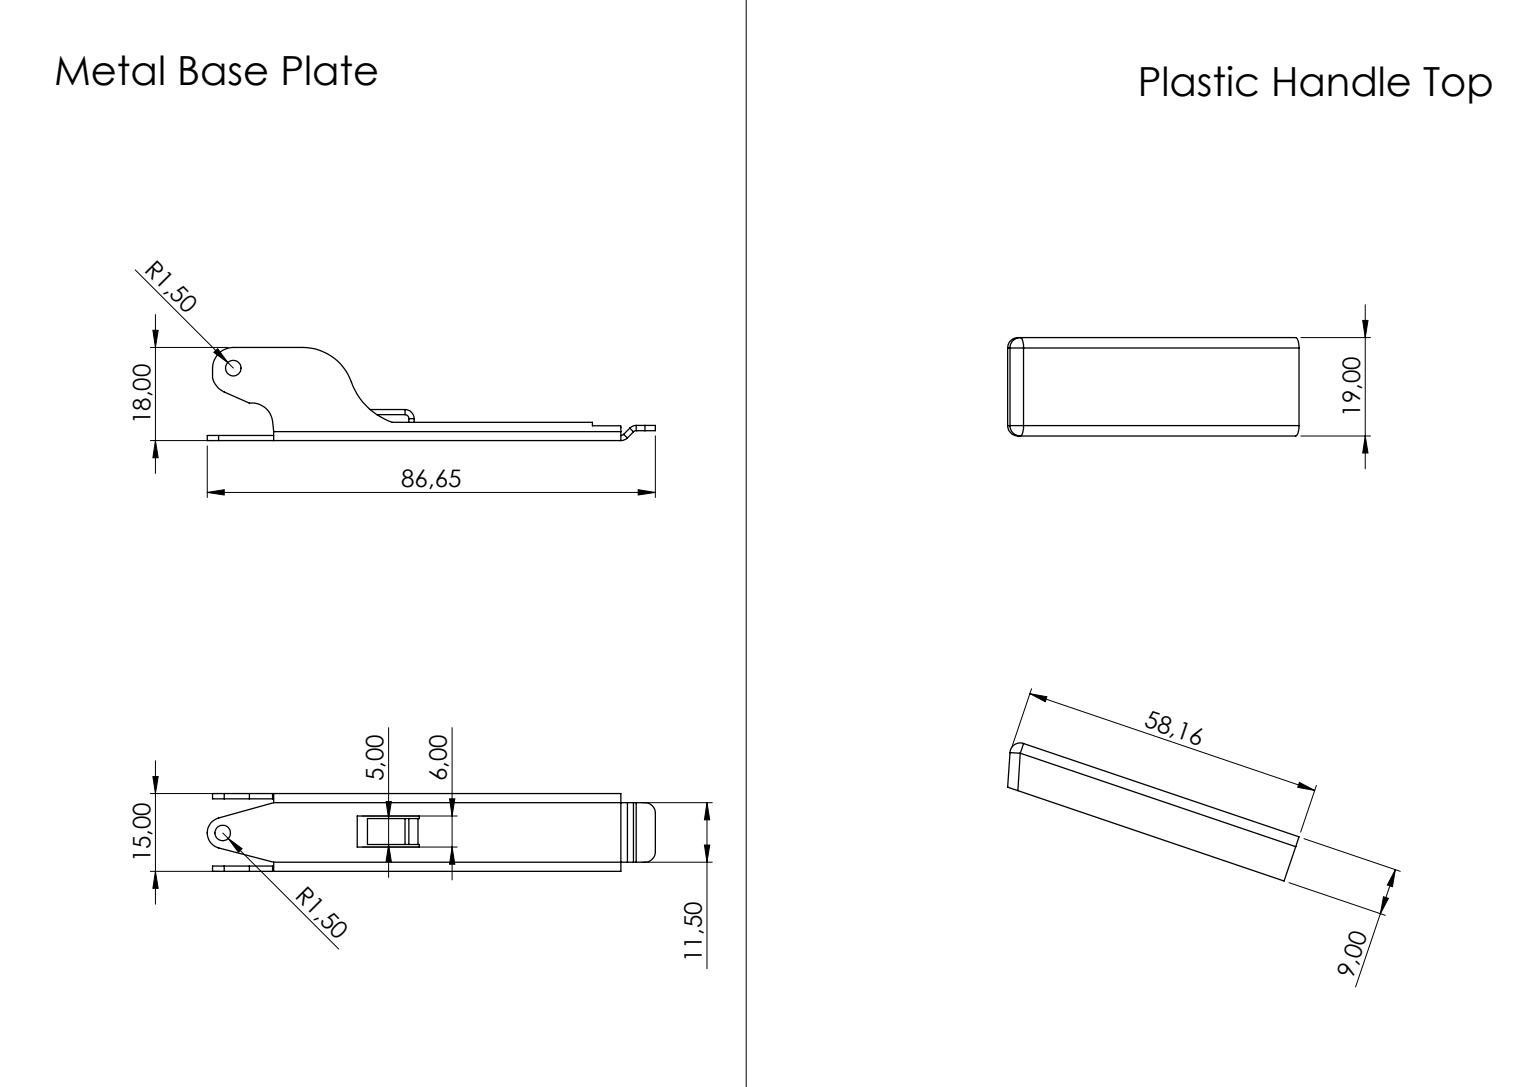
ISO-10303-21;
HEADER;
FILE_DESCRIPTION (('STEP AP214'),
    '1' );
FILE_NAME ('Plastic Handle Top.step',
    '2026-10-06T10:23:46',
    ( '' ),
    ( '' ),
    'SwSTEP 2.0',
    'SolidWorks 2020',
    '' );
FILE_SCHEMA (( 'AUTOMOTIVE_DESIGN' ));
ENDSEC;

DATA;
#49=EDGE_LOOP ( 'NONE', ( #5787, #14617, #11097, #246 ) ) ;
#69=FACE_OUTER_BOUND ( 'NONE', #11931, .T. ) ;
#71=VECTOR ( 'NONE', #6423, 1000.000000000000227 ) ;
#106=ADVANCED_FACE ( 'NONE', ( #10603 ), #18707, .F. ) ;
#219=ORIENTED_EDGE ( 'NONE', *, *, #5616, .T. ) ;
#246=ORIENTED_EDGE ( 'NONE', *, *, #17263, .T. ) ;
#258=ADVANCED_FACE ( 'NONE', ( #25369 ), #5308, .T. ) ;
#299=LINE ( 'NONE', #10238, #21343 ) ;
#343=CARTESIAN_POINT ( 'NONE',  ( 45.81606138205698642, -7.197381196808444237, -3.552044091124070491 ) ) ;
#348=EDGE_CURVE ( 'NONE', #23547, #5555, #499, .T. ) ;
#362=DIRECTION ( 'NONE',  ( -2.385244779468109755E-15, 1.000000000000000000, 0.000000000000000000 ) ) ;
#417=CARTESIAN_POINT ( 'NONE',  ( 30.81606138205696155, 1.773964314019527588, -3.427682652428149623 ) ) ;
#434=ORIENTED_EDGE ( 'NONE', *, *, #3015, .T. ) ;
#447=CARTESIAN_POINT ( 'NONE',  ( 3.816061382056971762, -5.229446354161006560, -9.573232046949398111 ) ) ;
#499=LINE ( 'NONE', #627, #16776 ) ;
#526=AXIS2_PLACEMENT_3D ( 'NONE', #704, #5104, #14630 ) ;
#534=STYLED_ITEM ( 'NONE', ( #16830 ), #19676 ) ;
#560=AXIS2_PLACEMENT_3D ( 'NONE', #2943, #9027, #8898 ) ;
#575=DIRECTION ( 'NONE',  ( 1.000000000000000000, 2.440719103442460911E-15, 1.328886038262200866E-15 ) ) ;
#616=LINE ( 'NONE', #20345, #10667 ) ;
#627=CARTESIAN_POINT ( 'NONE',  ( 29.71606138205698500, -6.548589660139427338, -8.069948661059612505 ) ) ;
#631=CARTESIAN_POINT ( 'NONE',  ( 28.81606138205695444, -23.19619402982950263, 47.16846523730000484 ) ) ;
#704=CARTESIAN_POINT ( 'NONE',  ( 45.81606138205697221, -4.589472609077215104, -6.350807634294793225 ) ) ;
#750=VECTOR ( 'NONE', #17336, 1000.000000000000227 ) ;
#847=ORIENTED_EDGE ( 'NONE', *, *, #24054, .T. ) ;
#862=AXIS2_PLACEMENT_3D ( 'NONE', #7436, #23134, #19536 ) ;
#868=VERTEX_POINT ( 'NONE', #20952 ) ;
#878=CIRCLE ( 'NONE', #9556, 2.000000000000000888 ) ;
#921=CYLINDRICAL_SURFACE ( 'NONE', #3999, 1.100000000000000311 ) ;
#955=FACE_OUTER_BOUND ( 'NONE', #12125, .T. ) ;
#971=SHAPE_REPRESENTATION_RELATIONSHIP ( 'NONE' , 'NONE' ,  #9445, #19676 ) ;
#988=DIRECTION ( 'NONE',  ( -4.040217218240261171E-16, -0.4425581086832399702, 0.8967398287344627850 ) ) ;
#1046=DIRECTION ( 'NONE',  ( -2.727049986597863807E-15, 0.7516416929448760387, 0.6595716529892418079 ) ) ;
#1144=DIRECTION ( 'NONE',  ( 2.727049986597864201E-15, -0.7516416929448760387, -0.6595716529892418079 ) ) ;
#1189=EDGE_CURVE ( 'NONE', #17007, #11300, #6517, .T. ) ;
#1223=PLANE ( 'NONE',  #24789 ) ;
#1237=ORIENTED_EDGE ( 'NONE', *, *, #24724, .T. ) ;
#1291=CARTESIAN_POINT ( 'NONE',  ( 46.91606138205697363, -29.47337283097070681, 44.07055847651734837 ) ) ;
#1309=( LENGTH_UNIT ( ) NAMED_UNIT ( * ) SI_UNIT ( .MILLI., .METRE. ) );
#1431=VECTOR ( 'NONE', #1046, 1000.000000000000000 ) ;
#1439=( NAMED_UNIT ( * ) SI_UNIT ( $, .STERADIAN. ) SOLID_ANGLE_UNIT ( ) );
#1466=ADVANCED_FACE ( 'NONE', ( #21311 ), #19623, .F. ) ;
#1703=DIRECTION ( 'NONE',  ( -1.000000000000000000, -2.411023719125726758E-15, -1.389056744264227588E-15 ) ) ;
#1720=DIRECTION ( 'NONE',  ( -1.000000000000000000, -2.556434596176347380E-15, -1.460819769243627131E-15 ) ) ;
#1767=ORIENTED_EDGE ( 'NONE', *, *, #23665, .F. ) ;
#1771=( LENGTH_UNIT ( ) NAMED_UNIT ( * ) SI_UNIT ( .MILLI., .METRE. ) );
#1792=LINE ( 'NONE', #17788, #13583 ) ;
#1807=AXIS2_PLACEMENT_3D ( 'NONE', #21939, #14085, #12169 ) ;
#1879=PLANE ( 'NONE',  #4650 ) ;
#1958=VERTEX_POINT ( 'NONE', #16654 ) ;
#1977=EDGE_LOOP ( 'NONE', ( #14482, #18335, #5715, #7299 ) ) ;
#2000=AXIS2_PLACEMENT_3D ( 'NONE', #9286, #12766, #22537 ) ;
#2001=EDGE_CURVE ( 'NONE', #5682, #24395, #7833, .T. ) ;
#2034=DIRECTION ( 'NONE',  ( -1.156482317317872465E-16, -0.4425581086832399702, 0.8967398287344626739 ) ) ;
#2126=DIRECTION ( 'NONE',  ( 1.156482317317872711E-16, 0.4425581086832400257, -0.8967398287344628960 ) ) ;
#2251=CARTESIAN_POINT ( 'NONE',  ( 28.81606138205696155, 0.8576245772853319238, -1.570935883000529332 ) ) ;
#2255=EDGE_LOOP ( 'NONE', ( #4585, #7218, #14724, #219 ) ) ;
#2277=EDGE_LOOP ( 'NONE', ( #12064, #434, #20219 ) ) ;
#2401=VERTEX_POINT ( 'NONE', #417 ) ;
#2435=AXIS2_PLACEMENT_3D ( 'NONE', #23279, #13502, #23400 ) ;
#2456=DIRECTION ( 'NONE',  ( 0.000000000000000000, 0.4425581086832397482, -0.8967398287344626739 ) ) ;
#2489=AXIS2_PLACEMENT_3D ( 'NONE', #19390, #23374, #13359 ) ;
#2494=DIRECTION ( 'NONE',  ( -1.786044098272412642E-16, -0.4425581086832399702, 0.8967398287344628960 ) ) ;
#2543=APPLICATION_CONTEXT ( 'automotive_design' ) ;
#2606=EDGE_LOOP ( 'NONE', ( #14663, #13840, #20351 ) ) ;
#2613=DIRECTION ( 'NONE',  ( -1.156482317317870739E-16, -0.4425581086832400257, 0.8967398287344628960 ) ) ;
#2618=CARTESIAN_POINT ( 'NONE',  ( 3.816061382056946449, 1.361611432489073570, -2.592146606185760316 ) ) ;
#2803=ORIENTED_EDGE ( 'NONE', *, *, #5814, .F. ) ;
#2813=ORIENTED_EDGE ( 'NONE', *, *, #19782, .F. ) ;
#2821=DIRECTION ( 'NONE',  ( -2.727049986597864201E-15, 0.7516416929448760387, 0.6595716529892418079 ) ) ;
#2824=FACE_OUTER_BOUND ( 'NONE', #2255, .T. ) ;
#2838=ORIENTED_EDGE ( 'NONE', *, *, #6174, .T. ) ;
#2924=EDGE_CURVE ( 'NONE', #12220, #11300, #22115, .T. ) ;
#2943=CARTESIAN_POINT ( 'NONE',  ( 47.81606138205695089, -23.19619402982945644, 47.16846523730003327 ) ) ;
#2950=LINE ( 'NONE', #24581, #21507 ) ;
#2969=VERTEX_POINT ( 'NONE', #12020 ) ;
#2972=CARTESIAN_POINT ( 'NONE',  ( 45.81606138205697221, -4.589472609077215104, -6.350807634294793225 ) ) ;
#2995=VECTOR ( 'NONE', #19543, 1000.000000000000227 ) ;
#3001=DIRECTION ( 'NONE',  ( 1.156482317317872711E-16, 0.4425581086832400257, -0.8967398287344628960 ) ) ;
#3015=EDGE_CURVE ( 'NONE', #3872, #13887, #6580, .T. ) ;
#3111=ADVANCED_FACE ( 'NONE', ( #2824 ), #6704, .T. ) ;
#3113=EDGE_CURVE ( 'NONE', #3872, #15753, #9022, .T. ) ;
#3213=DIRECTION ( 'NONE',  ( 2.776799322558808202E-15, -0.8967398287344627850, -0.4425581086832400257 ) ) ;
#3290=CARTESIAN_POINT ( 'NONE',  ( 47.81606138205697221, -29.47337283097070326, 44.07055847651734837 ) ) ;
#3426=( NAMED_UNIT ( * ) PLANE_ANGLE_UNIT ( ) SI_UNIT ( $, .RADIAN. ) );
#3490=ORIENTED_EDGE ( 'NONE', *, *, #19731, .F. ) ;
#3623=VECTOR ( 'NONE', #1720, 1000.000000000000000 ) ;
#3643=ORIENTED_EDGE ( 'NONE', *, *, #24491, .F. ) ;
#3644=LINE ( 'NONE', #21431, #13349 ) ;
#3650=DIRECTION ( 'NONE',  ( 2.727049986597864201E-15, -0.7516416929448760387, -0.6595716529892418079 ) ) ;
#3715=CARTESIAN_POINT ( 'NONE',  ( 45.81606138205697221, -4.589472609077215992, -6.350807634294793225 ) ) ;
#3781=AXIS2_PLACEMENT_3D ( 'NONE', #12203, #6014, #18125 ) ;
#3854=EDGE_CURVE ( 'NONE', #8842, #21203, #13959, .T. ) ;
#3866=DIRECTION ( 'NONE',  ( 1.000000000000000000, 2.452751524064190075E-15, 1.339444584486322859E-15 ) ) ;
#3872=VERTEX_POINT ( 'NONE', #5410 ) ;
#3908=CARTESIAN_POINT ( 'NONE',  ( 45.81606138205697931, -6.382952266546141118, -7.235923851661270945 ) ) ;
#3948=CYLINDRICAL_SURFACE ( 'NONE', #22674, 2.000000000000000888 ) ;
#3979=CARTESIAN_POINT ( 'NONE',  ( 30.81606138205697931, -4.589472609077251519, -6.350807634294812765 ) ) ;
#3994=ORIENTED_EDGE ( 'NONE', *, *, #7465, .F. ) ;
#3999=AXIS2_PLACEMENT_3D ( 'NONE', #7120, #14975, #22831 ) ;
#4000=ORIENTED_EDGE ( 'NONE', *, *, #23645, .T. ) ;
#4031=CARTESIAN_POINT ( 'NONE',  ( 28.81606138205695089, 1.394403967322826121, -2.658592958638802184 ) ) ;
#4078=PLANE ( 'NONE',  #21448 ) ;
#4099=ORIENTED_EDGE ( 'NONE', *, *, #4913, .F. ) ;
#4178=ORIENTED_EDGE ( 'NONE', *, *, #14604, .F. ) ;
#4203=CARTESIAN_POINT ( 'NONE',  ( 30.81606138205697931, -6.210967385200574675, -3.065230171572521645 ) ) ;
#4382=LINE ( 'NONE', #12626, #24258 ) ;
#4391=ADVANCED_FACE ( 'NONE', ( #24886 ), #16796, .F. ) ;
#4431=AXIS2_PLACEMENT_3D ( 'NONE', #2972, #8802, #18454 ) ;
#4512=CIRCLE ( 'NONE', #2435, 1.100000000000000311 ) ;
#4533=CARTESIAN_POINT ( 'NONE',  ( 45.81606138205695089, 1.361611432489176821, -2.592146606185703916 ) ) ;
#4570=VECTOR ( 'NONE', #11563, 1000.000000000000227 ) ;
#4585=ORIENTED_EDGE ( 'NONE', *, *, #5809, .T. ) ;
#4633=UNCERTAINTY_MEASURE_WITH_UNIT (LENGTH_MEASURE( 1.000000000000000082E-05 ), #1771, 'distance_accuracy_value', 'NONE');
#4640=ORIENTED_EDGE ( 'NONE', *, *, #17576, .F. ) ;
#4650=AXIS2_PLACEMENT_3D ( 'NONE', #15290, #5515, #15164 ) ;
#4717=PRODUCT_DEFINITION_FORMATION_WITH_SPECIFIED_SOURCE ( 'ANY', '', #11362, .NOT_KNOWN. ) ;
#4791=CARTESIAN_POINT ( 'NONE',  ( 3.816061382056972207, -3.863943790789065691, -7.177613496534135606 ) ) ;
#4913=EDGE_CURVE ( 'NONE', #868, #2401, #16899, .T. ) ;
#4966=EDGE_LOOP ( 'NONE', ( #17447, #12628, #13369, #10650 ) ) ;
#4984=DIRECTION ( 'NONE',  ( 1.000000000000000000, 2.440719103442461700E-15, 1.328886038262201260E-15 ) ) ;
#5024=AXIS2_PLACEMENT_3D ( 'NONE', #25467, #7595, #12106 ) ;
#5031=CARTESIAN_POINT ( 'NONE',  ( 2.480162969315272434E-14, -8.004447042669575296, -3.950346388939042885 ) ) ;
#5035=ORIENTED_EDGE ( 'NONE', *, *, #24912, .F. ) ;
#5104=DIRECTION ( 'NONE',  ( 1.493079894517851385E-15, 0.4425581086832399147, -0.8967398287344626739 ) ) ;
#5119=ORIENTED_EDGE ( 'NONE', *, *, #22759, .F. ) ;
#5125=ORIENTED_EDGE ( 'NONE', *, *, #5616, .F. ) ;
#5132=DIRECTION ( 'NONE',  ( 0.000000000000000000, -0.8967398287344627850, -0.4425581086832399702 ) ) ;
#5163=ORIENTED_EDGE ( 'NONE', *, *, #10385, .F. ) ;
#5200=FACE_OUTER_BOUND ( 'NONE', #18200, .T. ) ;
#5234=CARTESIAN_POINT ( 'NONE',  ( 45.81606138205695089, 1.773964314019564448, -3.427682652428129195 ) ) ;
#5308=PLANE ( 'NONE',  #13883 ) ;
#5352=ORIENTED_EDGE ( 'NONE', *, *, #6293, .T. ) ;
#5410=CARTESIAN_POINT ( 'NONE',  ( 47.81606138205697931, -4.589472609077211551, -6.350807634294790560 ) ) ;
#5422=ORIENTED_EDGE ( 'NONE', *, *, #23086, .F. ) ;
#5427=ORIENTED_EDGE ( 'NONE', *, *, #3113, .T. ) ;
#5515=DIRECTION ( 'NONE',  ( 6.109829820097539848E-16, -0.6595716529892418079, 0.7516416929448760387 ) ) ;
#5555=VERTEX_POINT ( 'NONE', #12516 ) ;
#5576=SHAPE_DEFINITION_REPRESENTATION ( #25327, #9445 ) ;
#5616=EDGE_CURVE ( 'NONE', #13887, #14165, #23652, .T. ) ;
#5677=ORIENTED_EDGE ( 'NONE', *, *, #20745, .T. ) ;
#5682=VERTEX_POINT ( 'NONE', #11946 ) ;
#5715=ORIENTED_EDGE ( 'NONE', *, *, #348, .T. ) ;
#5732=VECTOR ( 'NONE', #11228, 1000.000000000000000 ) ;
#5734=DIRECTION ( 'NONE',  ( 0.000000000000000000, 0.4425581086832399702, -0.8967398287344626739 ) ) ;
#5782=VECTOR ( 'NONE', #23672, 1000.000000000000000 ) ;
#5787=ORIENTED_EDGE ( 'NONE', *, *, #9395, .T. ) ;
#5809=EDGE_CURVE ( 'NONE', #14165, #19639, #14493, .T. ) ;
#5814=EDGE_CURVE ( 'NONE', #24859, #20881, #21850, .T. ) ;
#5834=FACE_OUTER_BOUND ( 'NONE', #13508, .T. ) ;
#5968=EDGE_LOOP ( 'NONE', ( #20132, #9383, #11486, #17134 ) ) ;
#5992=CARTESIAN_POINT ( 'NONE',  ( 30.81606138205697931, -3.863943790789087895, -7.177613496534175574 ) ) ;
#6012=DIRECTION ( 'NONE',  ( 0.000000000000000000, 0.8967398287344626739, 0.4425581086832399147 ) ) ;
#6014=DIRECTION ( 'NONE',  ( 1.000000000000000000, 2.490066548941357028E-15, 1.228895056384528999E-15 ) ) ;
#6033=CARTESIAN_POINT ( 'NONE',  ( 45.81606138205697931, -6.548589660139387369, -8.069948661059591188 ) ) ;
#6125=CARTESIAN_POINT ( 'NONE',  ( 45.81606138205697931, -30.45978664257862434, 43.58374455696579730 ) ) ;
#6174=EDGE_CURVE ( 'NONE', #24859, #17007, #3644, .T. ) ;
#6214=ADVANCED_FACE ( 'NONE', ( #16378 ), #12291, .T. ) ;
#6256=ORIENTED_EDGE ( 'NONE', *, *, #14050, .T. ) ;
#6293=EDGE_CURVE ( 'NONE', #21203, #12220, #22317, .T. ) ;
#6350=EDGE_CURVE ( 'NONE', #9234, #24670, #24355, .T. ) ;
#6354=ORIENTED_EDGE ( 'NONE', *, *, #2001, .T. ) ;
#6397=AXIS2_PLACEMENT_3D ( 'NONE', #21913, #8519, #18058 ) ;
#6417=EDGE_CURVE ( 'NONE', #3872, #5682, #24603, .T. ) ;
#6423=DIRECTION ( 'NONE',  ( -0.000000000000000000, -0.4425581086832399702, 0.8967398287344626739 ) ) ;
#6446=DIRECTION ( 'NONE',  ( 2.727049986597864201E-15, -0.7516416929448760387, -0.6595716529892418079 ) ) ;
#6464=AXIS2_PLACEMENT_3D ( 'NONE', #9572, #25251, #19726 ) ;
#6501=ORIENTED_EDGE ( 'NONE', *, *, #5814, .T. ) ;
#6517=LINE ( 'NONE', #16422, #18384 ) ;
#6580=CIRCLE ( 'NONE', #9890, 2.000000000000000000 ) ;
#6682=ORIENTED_EDGE ( 'NONE', *, *, #3854, .F. ) ;
#6704=PLANE ( 'NONE',  #15985 ) ;
#6738=DIRECTION ( 'NONE',  ( -1.156482317317870739E-16, -0.4425581086832400257, 0.8967398287344628960 ) ) ;
#6883=VERTEX_POINT ( 'NONE', #7078 ) ;
#7031=FACE_OUTER_BOUND ( 'NONE', #20181, .T. ) ;
#7075=EDGE_CURVE ( 'NONE', #13774, #2969, #9534, .T. ) ;
#7078=CARTESIAN_POINT ( 'NONE',  ( 45.81606138205698642, -5.575886420685123745, -6.837621553846354949 ) ) ;
#7108=CARTESIAN_POINT ( 'NONE',  ( 30.81606138205696155, 1.773964314019528477, -3.427682652428150067 ) ) ;
#7113=CARTESIAN_POINT ( 'NONE',  ( 47.81606138205695800, 0.4548210080410876599, -1.924399266538374009 ) ) ;
#7120=CARTESIAN_POINT ( 'NONE',  ( 45.81606138205697931, -6.548589660139387369, -8.069948661059591188 ) ) ;
#7135=EDGE_CURVE ( 'NONE', #5555, #20798, #11592, .T. ) ;
#7145=ORIENTED_EDGE ( 'NONE', *, *, #17263, .F. ) ;
#7163=DIRECTION ( 'NONE',  ( 1.156482317317870492E-16, 0.4425581086832399702, -0.8967398287344626739 ) ) ;
#7206=ORIENTED_EDGE ( 'NONE', *, *, #20424, .T. ) ;
#7215=CARTESIAN_POINT ( 'NONE',  ( 46.91606138205695231, -23.19619402982945644, 47.16846523730003327 ) ) ;
#7218=ORIENTED_EDGE ( 'NONE', *, *, #24491, .T. ) ;
#7299=ORIENTED_EDGE ( 'NONE', *, *, #9417, .F. ) ;
#7412=DIRECTION ( 'NONE',  ( 1.000000000000000000, 2.490066548941357423E-15, 1.228895056384527422E-15 ) ) ;
#7435=CARTESIAN_POINT ( 'NONE',  ( 29.71606138205696368, 0.06621141594066179414, 0.03267658921015577367 ) ) ;
#7436=CARTESIAN_POINT ( 'NONE',  ( 30.81606138205697221, -29.47337283097074234, 44.07055847651731995 ) ) ;
#7453=PLANE ( 'NONE',  #15618 ) ;
#7465=EDGE_CURVE ( 'NONE', #9234, #1958, #9990, .T. ) ;
#7472=( GEOMETRIC_REPRESENTATION_CONTEXT ( 3 ) GLOBAL_UNCERTAINTY_ASSIGNED_CONTEXT ( ( #12580 ) ) GLOBAL_UNIT_ASSIGNED_CONTEXT ( ( #1309, #19101, #1439 ) ) REPRESENTATION_CONTEXT ( 'NONE', 'WORKASPACE' ) );
#7549=LINE ( 'NONE', #15400, #3623 ) ;
#7595=DIRECTION ( 'NONE',  ( -1.786044098272412642E-16, -0.4425581086832399702, 0.8967398287344628960 ) ) ;
#7650=EDGE_LOOP ( 'NONE', ( #11210, #5427, #18516, #21243 ) ) ;
#7654=ORIENTED_EDGE ( 'NONE', *, *, #14473, .F. ) ;
#7695=EDGE_CURVE ( 'NONE', #868, #9234, #878, .T. ) ;
#7770=ADVANCED_FACE ( 'NONE', ( #22444 ), #10260, .F. ) ;
#7833=( BOUNDED_CURVE ( )  B_SPLINE_CURVE ( 3, ( #13430, #15352, #11376, #13182 ),
 .UNSPECIFIED., .F., .T. ) 
 B_SPLINE_CURVE_WITH_KNOTS ( ( 4, 4 ),
 ( 1.570796326794895004, 3.141592653589793116 ),
 .UNSPECIFIED. ) 
 CURVE ( )  GEOMETRIC_REPRESENTATION_ITEM ( )  RATIONAL_B_SPLINE_CURVE ( ( 1.000000000000000000, 0.8047378541243646044, 0.8047378541243646044, 1.000000000000000000 ) ) 
 REPRESENTATION_ITEM ( '' )  );
#7841=LINE ( 'NONE', #15304, #5782 ) ;
#7872=ORIENTED_EDGE ( 'NONE', *, *, #5809, .F. ) ;
#8002=CYLINDRICAL_SURFACE ( 'NONE', #23442, 2.000000000000000000 ) ;
#8024=DIRECTION ( 'NONE',  ( -1.000000000000000000, -1.497661361212515810E-15, -3.239770556388344395E-15 ) ) ;
#8072=ORIENTED_EDGE ( 'NONE', *, *, #12737, .F. ) ;
#8091=DIRECTION ( 'NONE',  ( -1.000000000000000000, -2.556434596176347380E-15, -1.460819769243627131E-15 ) ) ;
#8096=ORIENTED_EDGE ( 'NONE', *, *, #22081, .F. ) ;
#8228=AXIS2_PLACEMENT_3D ( 'NONE', #10761, #3001, #22848 ) ;
#8268=CIRCLE ( 'NONE', #2489, 2.000000000000000000 ) ;
#8324=DIRECTION ( 'NONE',  ( -1.000000000000000000, -2.556434596176347380E-15, -1.460819769243627131E-15 ) ) ;
#8372=DIRECTION ( 'NONE',  ( 2.792262043613788141E-15, -0.8967398287344626739, -0.4425581086832399147 ) ) ;
#8402=EDGE_CURVE ( 'NONE', #5555, #11300, #16808, .T. ) ;
#8419=ORIENTED_EDGE ( 'NONE', *, *, #14782, .F. ) ;
#8454=ORIENTED_EDGE ( 'NONE', *, *, #7135, .F. ) ;
#8519=DIRECTION ( 'NONE',  ( 1.000000000000000000, 2.452751524064188892E-15, 1.339444584486322859E-15 ) ) ;
#8530=CIRCLE ( 'NONE', #6464, 2.000000000000000000 ) ;
#8607=ORIENTED_EDGE ( 'NONE', *, *, #3854, .T. ) ;
#8645=FACE_OUTER_BOUND ( 'NONE', #49, .T. ) ;
#8802=DIRECTION ( 'NONE',  ( 1.000000000000000000, 2.490066548941357028E-15, 1.228895056384528999E-15 ) ) ;
#8842=VERTEX_POINT ( 'NONE', #24483 ) ;
#8847=VECTOR ( 'NONE', #23855, 1000.000000000000227 ) ;
#8859=FILL_AREA_STYLE ('',( #13773 ) ) ;
#8890=VERTEX_POINT ( 'NONE', #14842 ) ;
#8898=DIRECTION ( 'NONE',  ( -2.452751524064188892E-15, 1.000000000000000000, 0.000000000000000000 ) ) ;
#8899=ADVANCED_FACE ( 'NONE', ( #12928 ), #921, .F. ) ;
#8903=CARTESIAN_POINT ( 'NONE',  ( 28.81606138205698997, -6.548589660139430002, -8.069948661059614281 ) ) ;
#8938=EDGE_CURVE ( 'NONE', #868, #1958, #8530, .T. ) ;
#9022=CIRCLE ( 'NONE', #21755, 2.000000000000000000 ) ;
#9027=DIRECTION ( 'NONE',  ( 1.000000000000000000, 2.452751524064188892E-15, 1.339444584486322859E-15 ) ) ;
#9102=ADVANCED_FACE ( 'NONE', ( #18433 ), #18315, .F. ) ;
#9190=CIRCLE ( 'NONE', #526, 1.099999999999999867 ) ;
#9213=MECHANICAL_DESIGN_GEOMETRIC_PRESENTATION_REPRESENTATION('',(#534),#24807);
#9222=ORIENTED_EDGE ( 'NONE', *, *, #16436, .T. ) ;
#9234=VERTEX_POINT ( 'NONE', #19986 ) ;
#9277=CARTESIAN_POINT ( 'NONE',  ( 28.81606138205695444, -23.19619402982950263, 47.16846523730000484 ) ) ;
#9286=CARTESIAN_POINT ( 'NONE',  ( 0.000000000000000000, 0.000000000000000000, 0.000000000000000000 ) ) ;
#9322=PRESENTATION_STYLE_ASSIGNMENT (( #10985 ) ) ;
#9378=DIRECTION ( 'NONE',  ( 1.156482317317872465E-16, 0.4425581086832399702, -0.8967398287344626739 ) ) ;
#9383=ORIENTED_EDGE ( 'NONE', *, *, #7075, .F. ) ;
#9393=EDGE_LOOP ( 'NONE', ( #8607, #14361, #5163 ) ) ;
#9395=EDGE_CURVE ( 'NONE', #16417, #8890, #2950, .T. ) ;
#9417=EDGE_CURVE ( 'NONE', #12220, #5555, #16146, .T. ) ;
#9438=ORIENTED_EDGE ( 'NONE', *, *, #7135, .T. ) ;
#9445=SHAPE_REPRESENTATION ( 'Plastic Handle Top', ( #2000 ), #20728 ) ;
#9498=CARTESIAN_POINT ( 'NONE',  ( 30.81606138205697931, -5.823060841851313008, -8.896754523299021500 ) ) ;
#9525=AXIS2_PLACEMENT_3D ( 'NONE', #16163, #16541, #12585 ) ;
#9534=LINE ( 'NONE', #15440, #15445 ) ;
#9556=AXIS2_PLACEMENT_3D ( 'NONE', #14000, #19793, #20047 ) ;
#9572=CARTESIAN_POINT ( 'NONE',  ( 30.81606138205697931, -4.589472609077253296, -6.350807634294812765 ) ) ;
#9607=CARTESIAN_POINT ( 'NONE',  ( 30.81606138205698997, -30.45978664257865987, 43.58374455696577598 ) ) ;
#9755=CARTESIAN_POINT ( 'NONE',  ( 45.81606138205697931, -8.004447042669465162, -3.950346388938982045 ) ) ;
#9890=AXIS2_PLACEMENT_3D ( 'NONE', #14816, #18688, #16620 ) ;
#9960=CIRCLE ( 'NONE', #5024, 1.099999999999998312 ) ;
#9969=CARTESIAN_POINT ( 'NONE',  ( 45.81606138205697221, -31.26685248843962839, 43.18544225915087509 ) ) ;
#9990=CIRCLE ( 'NONE', #24358, 1.999999999999999778 ) ;
#10053=EDGE_CURVE ( 'NONE', #18026, #24670, #24929, .T. ) ;
#10056=ADVANCED_FACE ( 'NONE', ( #13754 ), #1879, .T. ) ;
#10059=AXIS2_PLACEMENT_3D ( 'NONE', #14746, #7412, #11149 ) ;
#10098=CARTESIAN_POINT ( 'NONE',  ( 28.81606138205696155, 0.8576245772853319238, -1.570935883000529332 ) ) ;
#10149=CARTESIAN_POINT ( 'NONE',  ( 28.81606138205695444, -23.19619402982950263, 47.16846523730000484 ) ) ;
#10238=CARTESIAN_POINT ( 'NONE',  ( 45.81606138205697931, -5.229446354160903532, -9.573232046949343044 ) ) ;
#10253=EDGE_LOOP ( 'NONE', ( #5035, #11003, #23694, #3643 ) ) ;
#10260=SPHERICAL_SURFACE ( 'NONE', #3781, 1.100000000000000089 ) ;
#10263=ORIENTED_EDGE ( 'NONE', *, *, #6350, .T. ) ;
#10316=DIRECTION ( 'NONE',  ( 1.156482317317871478E-16, 0.4425581086832399702, -0.8967398287344626739 ) ) ;
#10349=FILL_AREA_STYLE_COLOUR ( '', #17355 ) ;
#10370=ORIENTED_EDGE ( 'NONE', *, *, #18072, .F. ) ;
#10385=EDGE_CURVE ( 'NONE', #8842, #6883, #9190, .T. ) ;
#10387=CARTESIAN_POINT ( 'NONE',  ( 3.816061382056966433, -4.589472609077318133, -6.350807634294847404 ) ) ;
#10480=ORIENTED_EDGE ( 'NONE', *, *, #6293, .F. ) ;
#10487=FACE_OUTER_BOUND ( 'NONE', #10973, .T. ) ;
#10495=DIRECTION ( 'NONE',  ( 0.000000000000000000, -0.8967398287344626739, -0.4425581086832399147 ) ) ;
#10581=DIRECTION ( 'NONE',  ( 0.000000000000000000, -0.6595716529892419189, 0.7516416929448759277 ) ) ;
#10603=FACE_OUTER_BOUND ( 'NONE', #9393, .T. ) ;
#10650=ORIENTED_EDGE ( 'NONE', *, *, #17841, .F. ) ;
#10653=ORIENTED_EDGE ( 'NONE', *, *, #8402, .F. ) ;
#10667=VECTOR ( 'NONE', #8372, 1000.000000000000227 ) ;
#10679=AXIS2_PLACEMENT_3D ( 'NONE', #3715, #15570, #25084 ) ;
#10712=DIRECTION ( 'NONE',  ( 0.000000000000000000, 0.6595716529892415858, -0.7516416929448761497 ) ) ;
#10738=SURFACE_STYLE_FILL_AREA ( #18971 ) ;
#10761=CARTESIAN_POINT ( 'NONE',  ( 30.81606138205697931, -6.210967385200574675, -3.065230171572521645 ) ) ;
#10784=LINE ( 'NONE', #18635, #17333 ) ;
#10814=UNCERTAINTY_MEASURE_WITH_UNIT (LENGTH_MEASURE( 1.000000000000000082E-05 ), #24666, 'distance_accuracy_value', 'NONE');
#10852=ORIENTED_EDGE ( 'NONE', *, *, #23357, .T. ) ;
#10865=LINE ( 'NONE', #20781, #12440 ) ;
#10973=EDGE_LOOP ( 'NONE', ( #18626, #21487, #6501, #17423 ) ) ;
#10985=SURFACE_STYLE_USAGE ( .BOTH. , #23073 ) ;
#11003=ORIENTED_EDGE ( 'NONE', *, *, #6350, .F. ) ;
#11064=ORIENTED_EDGE ( 'NONE', *, *, #6174, .F. ) ;
#11090=DIRECTION ( 'NONE',  ( -2.727049986597863807E-15, 0.7516416929448760387, 0.6595716529892418079 ) ) ;
#11097=ORIENTED_EDGE ( 'NONE', *, *, #6417, .T. ) ;
#11149=DIRECTION ( 'NONE',  ( 0.000000000000000000, 0.4425581086832397482, -0.8967398287344626739 ) ) ;
#11169=SURFACE_STYLE_FILL_AREA ( #8859 ) ;
#11200=DIRECTION ( 'NONE',  ( 2.452751524064188892E-15, -1.000000000000000000, 0.000000000000000000 ) ) ;
#11210=ORIENTED_EDGE ( 'NONE', *, *, #6417, .F. ) ;
#11228=DIRECTION ( 'NONE',  ( -2.727049986597863807E-15, 0.7516416929448760387, 0.6595716529892418079 ) ) ;
#11300=VERTEX_POINT ( 'NONE', #19043 ) ;
#11305=CARTESIAN_POINT ( 'NONE',  ( 28.81606138205697576, -29.47337283097074589, 44.07055847651732705 ) ) ;
#11358=ORIENTED_EDGE ( 'NONE', *, *, #22759, .T. ) ;
#11362=PRODUCT ( 'Plastic Handle Top', 'Plastic Handle Top', '', ( #11380 ) ) ;
#11376=CARTESIAN_POINT ( 'NONE',  ( 46.98763425731077348, 1.773964314019564448, -3.427682652428131416 ) ) ;
#11380=PRODUCT_CONTEXT ( 'NONE', #21976, 'mechanical' ) ;
#11416=LINE ( 'NONE', #3290, #750 ) ;
#11486=ORIENTED_EDGE ( 'NONE', *, *, #20745, .F. ) ;
#11550=AXIS2_PLACEMENT_3D ( 'NONE', #6033, #23915, #20192 ) ;
#11563=DIRECTION ( 'NONE',  ( -1.156482317317870492E-16, -0.4425581086832399702, 0.8967398287344626739 ) ) ;
#11592=LINE ( 'NONE', #15182, #25181 ) ;
#11643=VECTOR ( 'NONE', #9378, 1000.000000000000227 ) ;
#11677=FACE_OUTER_BOUND ( 'NONE', #23537, .T. ) ;
#11825=CARTESIAN_POINT ( 'NONE',  ( 45.81606138205697221, -6.210967385200538260, -3.065230171572501661 ) ) ;
#11856=ADVANCED_FACE ( 'NONE', ( #7031 ), #1223, .F. ) ;
#11857=AXIS2_PLACEMENT_3D ( 'NONE', #23358, #3650, #13456 ) ;
#11898=DIRECTION ( 'NONE',  ( 1.000000000000000000, 2.490066548941357423E-15, 1.228895056384527422E-15 ) ) ;
#11931=EDGE_LOOP ( 'NONE', ( #15665, #7206, #14397, #4000 ) ) ;
#11940=LINE ( 'NONE', #9498, #22519 ) ;
#11945=VERTEX_POINT ( 'NONE', #18756 ) ;
#11946=CARTESIAN_POINT ( 'NONE',  ( 47.81606138205695800, 0.8576245772853805516, -1.570935883000508460 ) ) ;
#11949=DIRECTION ( 'NONE',  ( 6.109829820097539848E-16, -0.6595716529892418079, 0.7516416929448760387 ) ) ;
#11974=FACE_OUTER_BOUND ( 'NONE', #7650, .T. ) ;
#12018=STYLED_ITEM ( 'NONE', ( #9322 ), #17206 ) ;
#12020=CARTESIAN_POINT ( 'NONE',  ( 46.91606138205695231, -23.19619402982945644, 47.16846523730003327 ) ) ;
#12030=VECTOR ( 'NONE', #4984, 1000.000000000000000 ) ;
#12064=ORIENTED_EDGE ( 'NONE', *, *, #3113, .F. ) ;
#12106=DIRECTION ( 'NONE',  ( 0.000000000000000000, -0.8967398287344631180, -0.4425581086832393041 ) ) ;
#12125=EDGE_LOOP ( 'NONE', ( #18841, #20828, #24186, #5352 ) ) ;
#12169=DIRECTION ( 'NONE',  ( 0.000000000000000000, 0.6595716529892419189, -0.7516416929448759277 ) ) ;
#12203=CARTESIAN_POINT ( 'NONE',  ( 30.81606138205697931, -4.589472609077253296, -6.350807634294811876 ) ) ;
#12220=VERTEX_POINT ( 'NONE', #5992 ) ;
#12279=CARTESIAN_POINT ( 'NONE',  ( 30.81606138205697931, -4.589472609077253296, -6.350807634294811876 ) ) ;
#12291=CYLINDRICAL_SURFACE ( 'NONE', #1807, 2.000000000000000000 ) ;
#12323=EDGE_LOOP ( 'NONE', ( #25025, #20469, #10370, #10480 ) ) ;
#12395=ADVANCED_FACE ( 'NONE', ( #5200 ), #20275, .T. ) ;
#12440=VECTOR ( 'NONE', #14973, 1000.000000000000000 ) ;
#12516=CARTESIAN_POINT ( 'NONE',  ( 29.71606138205697789, -4.589472609077254184, -6.350807634294812765 ) ) ;
#12531=CARTESIAN_POINT ( 'NONE',  ( 45.81606138205697221, -4.589472609077215104, -6.350807634294792337 ) ) ;
#12580=UNCERTAINTY_MEASURE_WITH_UNIT (LENGTH_MEASURE( 1.000000000000000082E-05 ), #1309, 'distance_accuracy_value', 'NONE');
#12585=DIRECTION ( 'NONE',  ( 0.000000000000000000, -0.8967398287344631180, -0.4425581086832393041 ) ) ;
#12626=CARTESIAN_POINT ( 'NONE',  ( 2.230251030284979743E-14, -5.575886420685237432, -6.837621553846413569 ) ) ;
#12628=ORIENTED_EDGE ( 'NONE', *, *, #20424, .F. ) ;
#12670=DIRECTION ( 'NONE',  ( -1.000000000000000000, -4.029870553924695461E-16, 4.592402829583201910E-16 ) ) ;
#12726=CARTESIAN_POINT ( 'NONE',  ( 45.81606138205697931, -6.382952266546142006, -7.235923851661271833 ) ) ;
#12737=EDGE_CURVE ( 'NONE', #13774, #17582, #20994, .T. ) ;
#12766=DIRECTION ( 'NONE',  ( 0.000000000000000000, 0.000000000000000000, 1.000000000000000000 ) ) ;
#12767=VERTEX_POINT ( 'NONE', #18562 ) ;
#12832=SPHERICAL_SURFACE ( 'NONE', #10059, 2.000000000000000000 ) ;
#12901=DIRECTION ( 'NONE',  ( 0.000000000000000000, 0.4425581086832399702, -0.8967398287344626739 ) ) ;
#12928=FACE_OUTER_BOUND ( 'NONE', #13130, .T. ) ;
#13081=CLOSED_SHELL ( 'NONE', ( #23615, #21165, #258, #16386, #3111, #25118, #6214, #24284, #12395, #16817, #23650, #21617, #25042, #11856, #9102, #19692, #10056, #1466, #8899, #13393, #106, #16787, #7770, #4391 ) ) ;
#13104=VECTOR ( 'NONE', #7163, 1000.000000000000227 ) ;
#13130=EDGE_LOOP ( 'NONE', ( #5677, #17569, #847, #6682 ) ) ;
#13182=CARTESIAN_POINT ( 'NONE',  ( 45.81606138205695089, 1.773964314019564448, -3.427682652428129195 ) ) ;
#13349=VECTOR ( 'NONE', #1703, 1000.000000000000000 ) ;
#13359=DIRECTION ( 'NONE',  ( 3.469446951953614189E-15, -1.000000000000000000, 0.000000000000000000 ) ) ;
#13369=ORIENTED_EDGE ( 'NONE', *, *, #24646, .T. ) ;
#13393=ADVANCED_FACE ( 'NONE', ( #10487 ), #25445, .F. ) ;
#13396=ORIENTED_EDGE ( 'NONE', *, *, #22081, .T. ) ;
#13430=CARTESIAN_POINT ( 'NONE',  ( 47.81606138205695800, 0.8576245772853805516, -1.570935883000508460 ) ) ;
#13456=DIRECTION ( 'NONE',  ( 0.000000000000000000, 0.6595716529892420299, -0.7516416929448758166 ) ) ;
#13475=ORIENTED_EDGE ( 'NONE', *, *, #7695, .F. ) ;
#13502=DIRECTION ( 'NONE',  ( -1.000000000000000000, -2.440719103442460911E-15, -1.328886038262200866E-15 ) ) ;
#13508=EDGE_LOOP ( 'NONE', ( #13475, #15944, #3994 ) ) ;
#13583=VECTOR ( 'NONE', #3866, 1000.000000000000000 ) ;
#13602=CARTESIAN_POINT ( 'NONE',  ( 30.81606138205697931, 1.361611432489137741, -2.592146606185725677 ) ) ;
#13623=VERTEX_POINT ( 'NONE', #2251 ) ;
#13672=CARTESIAN_POINT ( 'NONE',  ( 28.81606138205695444, -23.19619402982950263, 47.16846523730000484 ) ) ;
#13729=ORIENTED_EDGE ( 'NONE', *, *, #10053, .T. ) ;
#13754=FACE_OUTER_BOUND ( 'NONE', #12323, .T. ) ;
#13773=FILL_AREA_STYLE_COLOUR ( '', #24403 ) ;
#13774=VERTEX_POINT ( 'NONE', #24763 ) ;
#13788=CARTESIAN_POINT ( 'NONE',  ( -3.287286993713738101E-16, 0.06621141594058931046, 0.03267658921011617340 ) ) ;
#13840=ORIENTED_EDGE ( 'NONE', *, *, #8402, .T. ) ;
#13883=AXIS2_PLACEMENT_3D ( 'NONE', #13672, #17409, #15343 ) ;
#13887=VERTEX_POINT ( 'NONE', #3908 ) ;
#13959=CIRCLE ( 'NONE', #10679, 1.100000000000000311 ) ;
#14000=CARTESIAN_POINT ( 'NONE',  ( 30.81606138205697931, -4.589472609077253296, -6.350807634294811876 ) ) ;
#14050=EDGE_CURVE ( 'NONE', #2401, #13623, #25204, .T. ) ;
#14085=DIRECTION ( 'NONE',  ( 2.727049986597864201E-15, -0.7516416929448760387, -0.6595716529892418079 ) ) ;
#14101=DIRECTION ( 'NONE',  ( 2.727049986597864201E-15, -0.7516416929448760387, -0.6595716529892418079 ) ) ;
#14123=ORIENTED_EDGE ( 'NONE', *, *, #1189, .F. ) ;
#14124=DIRECTION ( 'NONE',  ( 0.000000000000000000, -0.7516416929448760387, -0.6595716529892418079 ) ) ;
#14154=LINE ( 'NONE', #343, #71 ) ;
#14165=VERTEX_POINT ( 'NONE', #9969 ) ;
#14254=DIRECTION ( 'NONE',  ( 0.000000000000000000, 0.4425581086832399702, -0.8967398287344626739 ) ) ;
#14293=CARTESIAN_POINT ( 'NONE',  ( 3.816061382056966433, -4.589472609077318133, -6.350807634294847404 ) ) ;
#14317=CARTESIAN_POINT ( 'NONE',  ( 46.91606138205695231, 0.8576245772853769989, -1.570935883000508460 ) ) ;
#14331=CARTESIAN_POINT ( 'NONE',  ( 30.81606138205696155, 1.773964314019527588, -3.427682652428149623 ) ) ;
#14352=EDGE_LOOP ( 'NONE', ( #19142, #19796, #10653, #9438 ) ) ;
#14361=ORIENTED_EDGE ( 'NONE', *, *, #22532, .T. ) ;
#14388=LINE ( 'NONE', #10149, #25043 ) ;
#14397=ORIENTED_EDGE ( 'NONE', *, *, #4913, .T. ) ;
#14452=ORIENTED_EDGE ( 'NONE', *, *, #10053, .F. ) ;
#14473=EDGE_CURVE ( 'NONE', #20798, #17007, #9960, .T. ) ;
#14482=ORIENTED_EDGE ( 'NONE', *, *, #18072, .T. ) ;
#14493=LINE ( 'NONE', #20299, #25108 ) ;
#14604=EDGE_CURVE ( 'NONE', #6883, #24859, #14154, .T. ) ;
#14617=ORIENTED_EDGE ( 'NONE', *, *, #19731, .T. ) ;
#14630=DIRECTION ( 'NONE',  ( 0.000000000000000000, 0.8967398287344625629, 0.4425581086832402478 ) ) ;
#14663=ORIENTED_EDGE ( 'NONE', *, *, #9417, .T. ) ;
#14724=ORIENTED_EDGE ( 'NONE', *, *, #17841, .T. ) ;
#14746=CARTESIAN_POINT ( 'NONE',  ( 45.81606138205697221, -4.589472609077215104, -6.350807634294793225 ) ) ;
#14782=EDGE_CURVE ( 'NONE', #11945, #23547, #22634, .T. ) ;
#14816=CARTESIAN_POINT ( 'NONE',  ( 45.81606138205697221, -4.589472609077215992, -6.350807634294792337 ) ) ;
#14839=CIRCLE ( 'NONE', #18151, 1.999999999999997113 ) ;
#14842=CARTESIAN_POINT ( 'NONE',  ( 47.81606138205697221, -29.47337283097070326, 44.07055847651734837 ) ) ;
#14885=SURFACE_STYLE_USAGE ( .BOTH. , #22877 ) ;
#14899=VECTOR ( 'NONE', #1144, 1000.000000000000000 ) ;
#14973=DIRECTION ( 'NONE',  ( -1.156482317317871478E-16, -0.4425581086832399147, 0.8967398287344627850 ) ) ;
#14975=DIRECTION ( 'NONE',  ( -2.727049986597863807E-15, 0.7516416929448760387, 0.6595716529892418079 ) ) ;
#15057=DIRECTION ( 'NONE',  ( 2.792262043613788141E-15, -0.8967398287344626739, -0.4425581086832399147 ) ) ;
#15063=DIRECTION ( 'NONE',  ( 2.792262043613788535E-15, -0.8967398287344626739, -0.4425581086832399147 ) ) ;
#15130=DIRECTION ( 'NONE',  ( -2.365532012695645428E-15, 1.000000000000000000, 0.000000000000000000 ) ) ;
#15164=DIRECTION ( 'NONE',  ( 0.000000000000000000, -0.7516416929448760387, -0.6595716529892418079 ) ) ;
#15173=CARTESIAN_POINT ( 'NONE',  ( 45.81606138205697221, -3.863943790789048816, -7.177613496534156035 ) ) ;
#15182=CARTESIAN_POINT ( 'NONE',  ( 29.71606138205697789, -6.210967385200577340, -3.065230171572522977 ) ) ;
#15290=CARTESIAN_POINT ( 'NONE',  ( 3.816061382056972207, -5.823060841851324554, -8.896754523299009065 ) ) ;
#15304=CARTESIAN_POINT ( 'NONE',  ( 45.81606138205695089, -5.823060841851306790, -8.896754523299028605 ) ) ;
#15343=DIRECTION ( 'NONE',  ( 0.000000000000000000, -0.8967398287344626739, -0.4425581086832399147 ) ) ;
#15352=CARTESIAN_POINT ( 'NONE',  ( 47.81606138205695800, 1.394403967322872306, -2.658592958638780424 ) ) ;
#15400=CARTESIAN_POINT ( 'NONE',  ( 28.81606138205695444, -23.19619402982950263, 47.16846523730000484 ) ) ;
#15411=DIRECTION ( 'NONE',  ( -0.000000000000000000, 0.7516416929448760387, 0.6595716529892418079 ) ) ;
#15440=CARTESIAN_POINT ( 'NONE',  ( 46.91606138205695942, 0.06621141594070373282, 0.03267658921017869283 ) ) ;
#15445=VECTOR ( 'NONE', #17515, 1000.000000000000227 ) ;
#15570=DIRECTION ( 'NONE',  ( -2.727049986597863807E-15, 0.7516416929448760387, 0.6595716529892418079 ) ) ;
#15618=AXIS2_PLACEMENT_3D ( 'NONE', #9277, #16861, #11200 ) ;
#15665=ORIENTED_EDGE ( 'NONE', *, *, #19863, .T. ) ;
#15715=FACE_OUTER_BOUND ( 'NONE', #18324, .T. ) ;
#15753=VERTEX_POINT ( 'NONE', #24106 ) ;
#15944=ORIENTED_EDGE ( 'NONE', *, *, #8938, .T. ) ;
#15980=CARTESIAN_POINT ( 'NONE',  ( 30.81606138205697931, -4.589472609077253296, -6.350807634294811876 ) ) ;
#15985=AXIS2_PLACEMENT_3D ( 'NONE', #5031, #3213, #12901 ) ;
#16004=CARTESIAN_POINT ( 'NONE',  ( 28.81606138205697576, -29.47337283097074945, 44.07055847651731995 ) ) ;
#16040=ORIENTED_EDGE ( 'NONE', *, *, #14782, .T. ) ;
#16091=DIRECTION ( 'NONE',  ( 1.000000000000000000, 2.490066548941357423E-15, 1.228895056384528013E-15 ) ) ;
#16115=LINE ( 'NONE', #23969, #23014 ) ;
#16146=CIRCLE ( 'NONE', #24781, 1.100000000000000311 ) ;
#16163=CARTESIAN_POINT ( 'NONE',  ( 45.81606138205696510, -29.47337283097071037, 44.07055847651734837 ) ) ;
#16168=EDGE_CURVE ( 'NONE', #18026, #13623, #21785, .T. ) ;
#16274=LINE ( 'NONE', #2618, #19754 ) ;
#16378=FACE_OUTER_BOUND ( 'NONE', #23258, .T. ) ;
#16386=ADVANCED_FACE ( 'NONE', ( #8645 ), #20612, .T. ) ;
#16387=AXIS2_PLACEMENT_3D ( 'NONE', #3979, #19190, #21370 ) ;
#16417=VERTEX_POINT ( 'NONE', #17004 ) ;
#16422=CARTESIAN_POINT ( 'NONE',  ( 30.81606138205698997, -7.197381196808482429, -3.552044091124089142 ) ) ;
#16436=EDGE_CURVE ( 'NONE', #2969, #20881, #24837, .T. ) ;
#16491=CARTESIAN_POINT ( 'NONE',  ( 46.46042646344656646, 1.361611432489177265, -2.592146606185704805 ) ) ;
#16541=DIRECTION ( 'NONE',  ( -1.786044098272412642E-16, -0.4425581086832399702, 0.8967398287344628960 ) ) ;
#16620=DIRECTION ( 'NONE',  ( 0.000000000000000000, 0.8967398287344631180, 0.4425581086832395261 ) ) ;
#16622=CARTESIAN_POINT ( 'NONE',  ( 46.91606138205695231, 1.152853241805996021, -2.169147274601560760 ) ) ;
#16654=CARTESIAN_POINT ( 'NONE',  ( 30.81606138205698642, -6.382952266546177533, -7.235923851661291373 ) ) ;
#16694=DIRECTION ( 'NONE',  ( -1.000000000000000000, -2.452751524064188892E-15, -1.339444584486322859E-15 ) ) ;
#16776=VECTOR ( 'NONE', #6446, 1000.000000000000000 ) ;
#16787=ADVANCED_FACE ( 'NONE', ( #955 ), #18615, .F. ) ;
#16796=CYLINDRICAL_SURFACE ( 'NONE', #8228, 1.099999999999999867 ) ;
#16808=CIRCLE ( 'NONE', #16387, 1.100000000000000089 ) ;
#16817=ADVANCED_FACE ( 'NONE', ( #20935 ), #12832, .T. ) ;
#16830=PRESENTATION_STYLE_ASSIGNMENT (( #14885 ) ) ;
#16861=DIRECTION ( 'NONE',  ( -1.000000000000000000, -2.452751524064188892E-15, -1.339444584486322859E-15 ) ) ;
#16899=LINE ( 'NONE', #7108, #24278 ) ;
#16951=CARTESIAN_POINT ( 'NONE',  ( 29.71606138205695657, -23.19619402982949907, 47.16846523730000484 ) ) ;
#17004=CARTESIAN_POINT ( 'NONE',  ( 47.81606138205695089, -23.19619402982945644, 47.16846523730003327 ) ) ;
#17007=VERTEX_POINT ( 'NONE', #9607 ) ;
#17092=( NAMED_UNIT ( * ) SI_UNIT ( $, .STERADIAN. ) SOLID_ANGLE_UNIT ( ) );
#17134=ORIENTED_EDGE ( 'NONE', *, *, #18913, .F. ) ;
#17206=MANIFOLD_SOLID_BREP ( 'Stock-MAS-155-1', #13081 ) ;
#17207=LINE ( 'NONE', #20943, #13104 ) ;
#17263=EDGE_CURVE ( 'NONE', #5682, #16417, #10865, .T. ) ;
#17333=VECTOR ( 'NONE', #18893, 1000.000000000000227 ) ;
#17336=DIRECTION ( 'NONE',  ( 1.156482317317870492E-16, 0.4425581086832399702, -0.8967398287344626739 ) ) ;
#17341=PRODUCT_DEFINITION ( 'UNKNOWN', '', #4717, #25202 ) ;
#17345=CARTESIAN_POINT ( 'NONE',  ( 28.81606138205695444, -23.19619402982950263, 47.16846523730000484 ) ) ;
#17355=COLOUR_RGB ( '', 0.08235294, 0.09019608, 0.10196078) ;
#17399=PLANE ( 'NONE',  #20563 ) ;
#17409=DIRECTION ( 'NONE',  ( -1.786044098272412642E-16, -0.4425581086832399702, 0.8967398287344627850 ) ) ;
#17423=ORIENTED_EDGE ( 'NONE', *, *, #18913, .T. ) ;
#17447=ORIENTED_EDGE ( 'NONE', *, *, #8938, .F. ) ;
#17469=DIRECTION ( 'NONE',  ( 2.776799322558808202E-15, -0.8967398287344627850, -0.4425581086832400257 ) ) ;
#17515=DIRECTION ( 'NONE',  ( -1.156482317317870492E-16, -0.4425581086832399702, 0.8967398287344626739 ) ) ;
#17569=ORIENTED_EDGE ( 'NONE', *, *, #12737, .T. ) ;
#17576=EDGE_CURVE ( 'NONE', #13623, #9234, #18683, .T. ) ;
#17582=VERTEX_POINT ( 'NONE', #20746 ) ;
#17726=DIRECTION ( 'NONE',  ( 0.000000000000000000, -0.8967398287344631180, -0.4425581086832393041 ) ) ;
#17788=CARTESIAN_POINT ( 'NONE',  ( 3.816061382056944229, 1.773964314019461419, -3.427682652428185595 ) ) ;
#17841=EDGE_CURVE ( 'NONE', #1958, #13887, #23918, .T. ) ;
#18002=ORIENTED_EDGE ( 'NONE', *, *, #7695, .T. ) ;
#18026=VERTEX_POINT ( 'NONE', #17345 ) ;
#18058=DIRECTION ( 'NONE',  ( -2.452751524064188892E-15, 1.000000000000000000, 0.000000000000000000 ) ) ;
#18072=EDGE_CURVE ( 'NONE', #12220, #12767, #11940, .T. ) ;
#18125=DIRECTION ( 'NONE',  ( 0.000000000000000000, 0.4425581086832403033, -0.8967398287344625629 ) ) ;
#18151=AXIS2_PLACEMENT_3D ( 'NONE', #24005, #2494, #17726 ) ;
#18200=EDGE_LOOP ( 'NONE', ( #25284, #3490, #20717, #5125 ) ) ;
#18284=AXIS2_PLACEMENT_3D ( 'NONE', #10387, #575, #15130 ) ;
#18315=PLANE ( 'NONE',  #6397 ) ;
#18317=( BOUNDED_CURVE ( )  B_SPLINE_CURVE ( 3, ( #13602, #19018, #19520, #21452 ),
 .UNSPECIFIED., .F., .T. ) 
 B_SPLINE_CURVE_WITH_KNOTS ( ( 4, 4 ),
 ( 1.794712260653050184E-16, 1.570796326794901221 ),
 .UNSPECIFIED. ) 
 CURVE ( )  GEOMETRIC_REPRESENTATION_ITEM ( )  RATIONAL_B_SPLINE_CURVE ( ( 1.000000000000000000, 0.8047378541243640493, 0.8047378541243640493, 1.000000000000000000 ) ) 
 REPRESENTATION_ITEM ( '' )  );
#18324=EDGE_LOOP ( 'NONE', ( #5119, #16040, #5422, #10852, #8072, #23901, #2813, #7145, #6354, #18477, #6256, #20908 ) ) ;
#18335=ORIENTED_EDGE ( 'NONE', *, *, #23086, .T. ) ;
#18381=CYLINDRICAL_SURFACE ( 'NONE', #11550, 1.999999999999999556 ) ;
#18384=VECTOR ( 'NONE', #14254, 1000.000000000000227 ) ;
#18400=CARTESIAN_POINT ( 'NONE',  ( 30.81606138205698286, -4.589472609077252407, -6.350807634294811876 ) ) ;
#18433=FACE_OUTER_BOUND ( 'NONE', #5968, .T. ) ;
#18454=DIRECTION ( 'NONE',  ( 0.000000000000000000, 0.4425581086832403033, -0.8967398287344625629 ) ) ;
#18477=ORIENTED_EDGE ( 'NONE', *, *, #23645, .F. ) ;
#18498=ORIENTED_EDGE ( 'NONE', *, *, #14050, .F. ) ;
#18516=ORIENTED_EDGE ( 'NONE', *, *, #19863, .F. ) ;
#18562=CARTESIAN_POINT ( 'NONE',  ( 30.81606138205697931, 1.361611432489137741, -2.592146606185725677 ) ) ;
#18615=CYLINDRICAL_SURFACE ( 'NONE', #18284, 1.100000000000000311 ) ;
#18626=ORIENTED_EDGE ( 'NONE', *, *, #10385, .T. ) ;
#18635=CARTESIAN_POINT ( 'NONE',  ( 30.81606138205698642, -8.004447042669500689, -3.950346388939002029 ) ) ;
#18654=VECTOR ( 'NONE', #10316, 1000.000000000000227 ) ;
#18683=LINE ( 'NONE', #8903, #14899 ) ;
#18688=DIRECTION ( 'NONE',  ( 1.512281363675413133E-17, 0.4425581086832396371, -0.8967398287344630070 ) ) ;
#18707=SPHERICAL_SURFACE ( 'NONE', #4431, 1.100000000000000089 ) ;
#18756=CARTESIAN_POINT ( 'NONE',  ( 29.71606138205695657, -23.19619402982949907, 47.16846523730000484 ) ) ;
#18841=ORIENTED_EDGE ( 'NONE', *, *, #2924, .T. ) ;
#18893=DIRECTION ( 'NONE',  ( 1.156482317317872465E-16, 0.4425581086832399702, -0.8967398287344626739 ) ) ;
#18913=EDGE_CURVE ( 'NONE', #20881, #8842, #17207, .T. ) ;
#18923=FACE_OUTER_BOUND ( 'NONE', #22297, .T. ) ;
#18971=FILL_AREA_STYLE ('',( #10349 ) ) ;
#19016=CARTESIAN_POINT ( 'NONE',  ( 30.81606138205697931, -31.26685248843966036, 43.18544225915084667 ) ) ;
#19018=CARTESIAN_POINT ( 'NONE',  ( 30.17169630066736019, 1.361611432489138185, -2.592146606185724789 ) ) ;
#19043=CARTESIAN_POINT ( 'NONE',  ( 30.81606138205698286, -5.575886420685161049, -6.837621553846377154 ) ) ;
#19101=( NAMED_UNIT ( * ) PLANE_ANGLE_UNIT ( ) SI_UNIT ( $, .RADIAN. ) );
#19142=ORIENTED_EDGE ( 'NONE', *, *, #14473, .T. ) ;
#19162=CARTESIAN_POINT ( 'NONE',  ( 28.81606138205695444, -23.19619402982950263, 47.16846523730000484 ) ) ;
#19190=DIRECTION ( 'NONE',  ( -1.156482317317872711E-16, -0.4425581086832400257, 0.8967398287344628960 ) ) ;
#19390=CARTESIAN_POINT ( 'NONE',  ( 45.81606138205697221, -4.589472609077215104, -6.350807634294792337 ) ) ;
#19478=DIRECTION ( 'NONE',  ( -1.000000000000000000, -2.440719103442460517E-15, -1.328886038262201063E-15 ) ) ;
#19520=CARTESIAN_POINT ( 'NONE',  ( 29.71606138205694947, 1.152853241805954498, -2.169147274601580744 ) ) ;
#19536=DIRECTION ( 'NONE',  ( 0.000000000000000000, -0.8967398287344635621, -0.4425581086832386379 ) ) ;
#19543=DIRECTION ( 'NONE',  ( 2.792262043613788535E-15, -0.8967398287344626739, -0.4425581086832399147 ) ) ;
#19623=CYLINDRICAL_SURFACE ( 'NONE', #11857, 1.099999999999999645 ) ;
#19639=VERTEX_POINT ( 'NONE', #19016 ) ;
#19676=ADVANCED_BREP_SHAPE_REPRESENTATION ( '', ( #17206, #2000 ), #20728 ) ;
#19692=ADVANCED_FACE ( 'NONE', ( #11677 ), #21450, .F. ) ;
#19704=FACE_OUTER_BOUND ( 'NONE', #4966, .T. ) ;
#19726=DIRECTION ( 'NONE',  ( 3.469446951953614189E-15, -1.000000000000000000, 0.000000000000000000 ) ) ;
#19731=EDGE_CURVE ( 'NONE', #8890, #3872, #11416, .T. ) ;
#19754=VECTOR ( 'NONE', #21139, 1000.000000000000000 ) ;
#19782=EDGE_CURVE ( 'NONE', #16417, #2969, #7549, .T. ) ;
#19793=DIRECTION ( 'NONE',  ( -2.727049986597864201E-15, 0.7516416929448760387, 0.6595716529892418079 ) ) ;
#19796=ORIENTED_EDGE ( 'NONE', *, *, #1189, .T. ) ;
#19797=CIRCLE ( 'NONE', #862, 2.000000000000000000 ) ;
#19863=EDGE_CURVE ( 'NONE', #24395, #15753, #299, .T. ) ;
#19928=AXIS2_PLACEMENT_3D ( 'NONE', #11825, #6738, #21727 ) ;
#19986=CARTESIAN_POINT ( 'NONE',  ( 28.81606138205698286, -4.589472609077256848, -6.350807634294814541 ) ) ;
#20047=DIRECTION ( 'NONE',  ( 0.000000000000000000, 0.6595716529892415858, -0.7516416929448760387 ) ) ;
#20132=ORIENTED_EDGE ( 'NONE', *, *, #16436, .F. ) ;
#20181=EDGE_LOOP ( 'NONE', ( #21300, #8419, #13396, #8454 ) ) ;
#20192=DIRECTION ( 'NONE',  ( 0.000000000000000000, -0.6595716529892415858, 0.7516416929448761497 ) ) ;
#20219=ORIENTED_EDGE ( 'NONE', *, *, #24646, .F. ) ;
#20275=CYLINDRICAL_SURFACE ( 'NONE', #20715, 2.000000000000000888 ) ;
#20299=CARTESIAN_POINT ( 'NONE',  ( 28.81606138205697931, -31.26685248843966747, 43.18544225915084667 ) ) ;
#20345=CARTESIAN_POINT ( 'NONE',  ( 29.71606138205695657, -23.19619402982949907, 47.16846523730000484 ) ) ;
#20351=ORIENTED_EDGE ( 'NONE', *, *, #2924, .F. ) ;
#20360=VECTOR ( 'NONE', #12670, 1000.000000000000000 ) ;
#20424=EDGE_CURVE ( 'NONE', #15753, #868, #16115, .T. ) ;
#20469=ORIENTED_EDGE ( 'NONE', *, *, #23357, .F. ) ;
#20563=AXIS2_PLACEMENT_3D ( 'NONE', #13788, #25356, #21388 ) ;
#20612=PLANE ( 'NONE',  #560 ) ;
#20635=DIRECTION ( 'NONE',  ( -2.727049986597864201E-15, 0.7516416929448760387, 0.6595716529892418079 ) ) ;
#20640=MECHANICAL_DESIGN_GEOMETRIC_PRESENTATION_REPRESENTATION('',(#12018),#7472);
#20657=CARTESIAN_POINT ( 'NONE',  ( 45.81606138205697221, -6.210967385200538260, -3.065230171572501661 ) ) ;
#20715=AXIS2_PLACEMENT_3D ( 'NONE', #20657, #2613, #10495 ) ;
#20717=ORIENTED_EDGE ( 'NONE', *, *, #24724, .F. ) ;
#20728=( GEOMETRIC_REPRESENTATION_CONTEXT ( 3 ) GLOBAL_UNCERTAINTY_ASSIGNED_CONTEXT ( ( #4633 ) ) GLOBAL_UNIT_ASSIGNED_CONTEXT ( ( #1771, #25337, #23416 ) ) REPRESENTATION_CONTEXT ( 'NONE', 'WORKASPACE' ) );
#20745=EDGE_CURVE ( 'NONE', #8842, #13774, #24970, .T. ) ;
#20746=CARTESIAN_POINT ( 'NONE',  ( 45.81606138205695089, 1.361611432489176821, -2.592146606185703916 ) ) ;
#20781=CARTESIAN_POINT ( 'NONE',  ( 47.81606138205695089, -23.19619402982945644, 47.16846523730003327 ) ) ;
#20798=VERTEX_POINT ( 'NONE', #23054 ) ;
#20828=ORIENTED_EDGE ( 'NONE', *, *, #23665, .T. ) ;
#20881=VERTEX_POINT ( 'NONE', #1291 ) ;
#20908=ORIENTED_EDGE ( 'NONE', *, *, #16168, .F. ) ;
#20935=FACE_OUTER_BOUND ( 'NONE', #2277, .T. ) ;
#20943=CARTESIAN_POINT ( 'NONE',  ( 46.91606138205698073, -6.210967385200536484, -3.065230171572500772 ) ) ;
#20952=CARTESIAN_POINT ( 'NONE',  ( 30.81606138205697931, -3.270329303098769014, -7.854091020184566396 ) ) ;
#20994=( BOUNDED_CURVE ( )  B_SPLINE_CURVE ( 3, ( #14317, #16622, #16491, #4533 ),
 .UNSPECIFIED., .F., .T. ) 
 B_SPLINE_CURVE_WITH_KNOTS ( ( 4, 4 ),
 ( 1.570796326794893227, 3.141592653589793116 ),
 .UNSPECIFIED. ) 
 CURVE ( )  GEOMETRIC_REPRESENTATION_ITEM ( )  RATIONAL_B_SPLINE_CURVE ( ( 1.000000000000000000, 0.8047378541243641603, 0.8047378541243641603, 1.000000000000000000 ) ) 
 REPRESENTATION_ITEM ( '' )  );
#21001=CARTESIAN_POINT ( 'NONE',  ( 30.81606138205697931, -4.589472609077253296, -6.350807634294812765 ) ) ;
#21139=DIRECTION ( 'NONE',  ( 1.000000000000000000, 2.440719103442460911E-15, 1.328886038262200866E-15 ) ) ;
#21165=ADVANCED_FACE ( 'NONE', ( #18923 ), #7453, .T. ) ;
#21200=CARTESIAN_POINT ( 'NONE',  ( 2.230251030284979743E-14, -7.197381196808558812, -3.552044091124126890 ) ) ;
#21203=VERTEX_POINT ( 'NONE', #15173 ) ;
#21243=ORIENTED_EDGE ( 'NONE', *, *, #2001, .F. ) ;
#21258=CARTESIAN_POINT ( 'NONE',  ( 29.71606138205696368, 0.8576245772853353655, -1.570935883000529332 ) ) ;
#21300=ORIENTED_EDGE ( 'NONE', *, *, #348, .F. ) ;
#21311=FACE_OUTER_BOUND ( 'NONE', #1977, .T. ) ;
#21324=AXIS2_PLACEMENT_3D ( 'NONE', #21200, #17469, #5734 ) ;
#21343=VECTOR ( 'NONE', #14101, 1000.000000000000000 ) ;
#21370=DIRECTION ( 'NONE',  ( 0.000000000000000000, 0.8967398287344627850, 0.4425581086832401922 ) ) ;
#21388=DIRECTION ( 'NONE',  ( 0.000000000000000000, 0.4425581086832399702, -0.8967398287344626739 ) ) ;
#21431=CARTESIAN_POINT ( 'NONE',  ( 1.291443647867872416E-14, -30.45978664257872381, 43.58374455696571914 ) ) ;
#21448=AXIS2_PLACEMENT_3D ( 'NONE', #447, #11949, #14124 ) ;
#21450=PLANE ( 'NONE',  #21324 ) ;
#21452=CARTESIAN_POINT ( 'NONE',  ( 29.71606138205696368, 0.8576245772853353655, -1.570935883000529332 ) ) ;
#21487=ORIENTED_EDGE ( 'NONE', *, *, #14604, .T. ) ;
#21507=VECTOR ( 'NONE', #15063, 1000.000000000000227 ) ;
#21617=ADVANCED_FACE ( 'NONE', ( #5834 ), #21672, .T. ) ;
#21672=SPHERICAL_SURFACE ( 'NONE', #21674, 2.000000000000000000 ) ;
#21674=AXIS2_PLACEMENT_3D ( 'NONE', #12279, #11898, #2456 ) ;
#21727=DIRECTION ( 'NONE',  ( 0.000000000000000000, -0.8967398287344625629, -0.4425581086832402478 ) ) ;
#21755=AXIS2_PLACEMENT_3D ( 'NONE', #12531, #11090, #10581 ) ;
#21785=LINE ( 'NONE', #631, #18654 ) ;
#21850=CIRCLE ( 'NONE', #9525, 1.099999999999998312 ) ;
#21913=CARTESIAN_POINT ( 'NONE',  ( 46.91606138205695231, -23.19619402982945644, 47.16846523730003327 ) ) ;
#21933=ORIENTED_EDGE ( 'NONE', *, *, #16168, .T. ) ;
#21939=CARTESIAN_POINT ( 'NONE',  ( 30.81606138205698642, -6.548589660139424673, -8.069948661059610728 ) ) ;
#21976=APPLICATION_CONTEXT ( 'automotive_design' ) ;
#22081=EDGE_CURVE ( 'NONE', #11945, #20798, #616, .T. ) ;
#22115=CIRCLE ( 'NONE', #24155, 1.100000000000000311 ) ;
#22297=EDGE_LOOP ( 'NONE', ( #24450, #10263, #14452, #21933 ) ) ;
#22317=LINE ( 'NONE', #4791, #20360 ) ;
#22444=FACE_OUTER_BOUND ( 'NONE', #2606, .T. ) ;
#22519=VECTOR ( 'NONE', #15411, 1000.000000000000000 ) ;
#22532=EDGE_CURVE ( 'NONE', #21203, #6883, #4512, .T. ) ;
#22537=DIRECTION ( 'NONE',  ( 1.000000000000000000, 0.000000000000000000, 0.000000000000000000 ) ) ;
#22634=LINE ( 'NONE', #7435, #11643 ) ;
#22674=AXIS2_PLACEMENT_3D ( 'NONE', #4203, #2126, #6012 ) ;
#22742=EDGE_LOOP ( 'NONE', ( #8096, #11358, #13729, #24595, #7872, #1237, #23281, #22864, #9222, #2803, #2838, #7654 ) ) ;
#22759=EDGE_CURVE ( 'NONE', #11945, #18026, #14388, .T. ) ;
#22831=DIRECTION ( 'NONE',  ( 0.000000000000000000, -0.6595716529892415858, 0.7516416929448761497 ) ) ;
#22848=DIRECTION ( 'NONE',  ( 0.000000000000000000, 0.8967398287344625629, 0.4425581086832402478 ) ) ;
#22864=ORIENTED_EDGE ( 'NONE', *, *, #19782, .T. ) ;
#22877=SURFACE_SIDE_STYLE ('',( #11169 ) ) ;
#23014=VECTOR ( 'NONE', #19478, 1000.000000000000000 ) ;
#23054=CARTESIAN_POINT ( 'NONE',  ( 29.71606138205697434, -29.47337283097074234, 44.07055847651732705 ) ) ;
#23073=SURFACE_SIDE_STYLE ('',( #10738 ) ) ;
#23086=EDGE_CURVE ( 'NONE', #12767, #23547, #18317, .T. ) ;
#23134=DIRECTION ( 'NONE',  ( -1.786044098272412642E-16, -0.4425581086832399702, 0.8967398287344628960 ) ) ;
#23258=EDGE_LOOP ( 'NONE', ( #4099, #18002, #4640, #18498 ) ) ;
#23279=CARTESIAN_POINT ( 'NONE',  ( 45.81606138205697221, -4.589472609077215992, -6.350807634294792337 ) ) ;
#23281=ORIENTED_EDGE ( 'NONE', *, *, #9395, .F. ) ;
#23357=EDGE_CURVE ( 'NONE', #12767, #17582, #16274, .T. ) ;
#23358=CARTESIAN_POINT ( 'NONE',  ( 30.81606138205698642, -6.548589660139424673, -8.069948661059610728 ) ) ;
#23374=DIRECTION ( 'NONE',  ( -1.000000000000000000, -2.699773532888683051E-15, -2.369073068322443402E-15 ) ) ;
#23400=DIRECTION ( 'NONE',  ( 0.000000000000000000, 1.000000000000000000, 0.000000000000000000 ) ) ;
#23416=( NAMED_UNIT ( * ) SI_UNIT ( $, .STERADIAN. ) SOLID_ANGLE_UNIT ( ) );
#23442=AXIS2_PLACEMENT_3D ( 'NONE', #14293, #24185, #362 ) ;
#23537=EDGE_LOOP ( 'NONE', ( #11064, #4178, #1767, #14123 ) ) ;
#23547=VERTEX_POINT ( 'NONE', #21258 ) ;
#23615=ADVANCED_FACE ( 'NONE', ( #15715 ), #17399, .F. ) ;
#23645=EDGE_CURVE ( 'NONE', #2401, #24395, #1792, .T. ) ;
#23650=ADVANCED_FACE ( 'NONE', ( #19704 ), #8002, .T. ) ;
#23652=LINE ( 'NONE', #9755, #4570 ) ;
#23655=FACE_OUTER_BOUND ( 'NONE', #10253, .T. ) ;
#23665=EDGE_CURVE ( 'NONE', #11300, #6883, #4382, .T. ) ;
#23672=DIRECTION ( 'NONE',  ( 0.000000000000000000, -0.7516416929448760387, -0.6595716529892418079 ) ) ;
#23694=ORIENTED_EDGE ( 'NONE', *, *, #7465, .T. ) ;
#23850=CARTESIAN_POINT ( 'NONE',  ( 29.64448850680314607, 1.773964314019522925, -3.427682652428152288 ) ) ;
#23855=DIRECTION ( 'NONE',  ( -1.156482317317872465E-16, -0.4425581086832399702, 0.8967398287344626739 ) ) ;
#23901=ORIENTED_EDGE ( 'NONE', *, *, #7075, .T. ) ;
#23915=DIRECTION ( 'NONE',  ( -2.727049986597863807E-15, 0.7516416929448760387, 0.6595716529892418079 ) ) ;
#23918=LINE ( 'NONE', #12726, #12030 ) ;
#23969=CARTESIAN_POINT ( 'NONE',  ( 30.81606138205698286, -3.270329303098768126, -7.854091020184564620 ) ) ;
#24005=CARTESIAN_POINT ( 'NONE',  ( 45.81606138205696510, -29.47337283097071037, 44.07055847651734837 ) ) ;
#24054=EDGE_CURVE ( 'NONE', #17582, #21203, #7841, .T. ) ;
#24086=DIRECTION ( 'NONE',  ( -3.154042683594193641E-15, 0.000000000000000000, 1.000000000000000000 ) ) ;
#24106=CARTESIAN_POINT ( 'NONE',  ( 45.81606138205697221, -3.270329303098730822, -7.854091020184544192 ) ) ;
#24155=AXIS2_PLACEMENT_3D ( 'NONE', #15980, #8024, #24086 ) ;
#24185=DIRECTION ( 'NONE',  ( 1.000000000000000000, 2.440719103442460911E-15, 1.328886038262200866E-15 ) ) ;
#24186=ORIENTED_EDGE ( 'NONE', *, *, #22532, .F. ) ;
#24258=VECTOR ( 'NONE', #16091, 1000.000000000000000 ) ;
#24278=VECTOR ( 'NONE', #20635, 1000.000000000000000 ) ;
#24284=ADVANCED_FACE ( 'NONE', ( #11974 ), #18381, .T. ) ;
#24355=LINE ( 'NONE', #16004, #8847 ) ;
#24358=AXIS2_PLACEMENT_3D ( 'NONE', #18400, #988, #5132 ) ;
#24395=VERTEX_POINT ( 'NONE', #5234 ) ;
#24403=COLOUR_RGB ( '', 0.08235294, 0.09019608, 0.10196078) ;
#24410=VECTOR ( 'NONE', #15057, 1000.000000000000227 ) ;
#24450=ORIENTED_EDGE ( 'NONE', *, *, #17576, .T. ) ;
#24483=CARTESIAN_POINT ( 'NONE',  ( 46.91606138205697363, -4.589472609077213328, -6.350807634294790560 ) ) ;
#24491=EDGE_CURVE ( 'NONE', #19639, #1958, #10784, .T. ) ;
#24581=CARTESIAN_POINT ( 'NONE',  ( 47.81606138205695089, -23.19619402982945644, 47.16846523730003327 ) ) ;
#24595=ORIENTED_EDGE ( 'NONE', *, *, #24912, .T. ) ;
#24603=LINE ( 'NONE', #7113, #1431 ) ;
#24646=EDGE_CURVE ( 'NONE', #15753, #13887, #8268, .T. ) ;
#24666=( LENGTH_UNIT ( ) NAMED_UNIT ( * ) SI_UNIT ( .MILLI., .METRE. ) );
#24670=VERTEX_POINT ( 'NONE', #11305 ) ;
#24722=CARTESIAN_POINT ( 'NONE',  ( 46.91606138205698073, -6.548589660139384705, -8.069948661059589412 ) ) ;
#24724=EDGE_CURVE ( 'NONE', #14165, #8890, #14839, .T. ) ;
#24763=CARTESIAN_POINT ( 'NONE',  ( 46.91606138205695231, 0.8576245772853769989, -1.570935883000508460 ) ) ;
#24781=AXIS2_PLACEMENT_3D ( 'NONE', #21001, #2821, #10712 ) ;
#24784=DIRECTION ( 'NONE',  ( 2.452751524064188892E-15, -1.000000000000000000, 0.000000000000000000 ) ) ;
#24789=AXIS2_PLACEMENT_3D ( 'NONE', #16951, #16694, #24784 ) ;
#24807=( GEOMETRIC_REPRESENTATION_CONTEXT ( 3 ) GLOBAL_UNCERTAINTY_ASSIGNED_CONTEXT ( ( #10814 ) ) GLOBAL_UNIT_ASSIGNED_CONTEXT ( ( #24666, #3426, #17092 ) ) REPRESENTATION_CONTEXT ( 'NONE', 'WORKASPACE' ) );
#24837=LINE ( 'NONE', #7215, #24410 ) ;
#24859=VERTEX_POINT ( 'NONE', #6125 ) ;
#24886=FACE_OUTER_BOUND ( 'NONE', #14352, .T. ) ;
#24912=EDGE_CURVE ( 'NONE', #24670, #19639, #19797, .T. ) ;
#24929=LINE ( 'NONE', #19162, #2995 ) ;
#24970=LINE ( 'NONE', #24722, #5732 ) ;
#25025=ORIENTED_EDGE ( 'NONE', *, *, #24054, .F. ) ;
#25042=ADVANCED_FACE ( 'NONE', ( #23655 ), #3948, .T. ) ;
#25043=VECTOR ( 'NONE', #8091, 1000.000000000000000 ) ;
#25084=DIRECTION ( 'NONE',  ( 0.000000000000000000, -0.6595716529892415858, 0.7516416929448761497 ) ) ;
#25108=VECTOR ( 'NONE', #8324, 1000.000000000000000 ) ;
#25118=ADVANCED_FACE ( 'NONE', ( #69 ), #4078, .F. ) ;
#25181=VECTOR ( 'NONE', #2034, 1000.000000000000227 ) ;
#25202=PRODUCT_DEFINITION_CONTEXT ( 'detailed design', #2543, 'design' ) ;
#25204=( BOUNDED_CURVE ( )  B_SPLINE_CURVE ( 3, ( #14331, #23850, #4031, #10098 ),
 .UNSPECIFIED., .F., .T. ) 
 B_SPLINE_CURVE_WITH_KNOTS ( ( 4, 4 ),
 ( 1.794712260653053635E-16, 1.570796326794900333 ),
 .UNSPECIFIED. ) 
 CURVE ( )  GEOMETRIC_REPRESENTATION_ITEM ( )  RATIONAL_B_SPLINE_CURVE ( ( 1.000000000000000000, 0.8047378541243641603, 0.8047378541243641603, 1.000000000000000000 ) ) 
 REPRESENTATION_ITEM ( '' )  );
#25251=DIRECTION ( 'NONE',  ( -1.000000000000000000, -2.699773532888685417E-15, -2.369073068322446951E-15 ) ) ;
#25284=ORIENTED_EDGE ( 'NONE', *, *, #3015, .F. ) ;
#25327=PRODUCT_DEFINITION_SHAPE ( 'NONE', 'NONE',  #17341 ) ;
#25337=( NAMED_UNIT ( * ) PLANE_ANGLE_UNIT ( ) SI_UNIT ( $, .RADIAN. ) );
#25356=DIRECTION ( 'NONE',  ( 2.776799322558808202E-15, -0.8967398287344627850, -0.4425581086832400257 ) ) ;
#25369=FACE_OUTER_BOUND ( 'NONE', #22742, .T. ) ;
#25445=CYLINDRICAL_SURFACE ( 'NONE', #19928, 1.099999999999999867 ) ;
#25467=CARTESIAN_POINT ( 'NONE',  ( 30.81606138205697221, -29.47337283097074234, 44.07055847651731995 ) ) ;
ENDSEC;
END-ISO-10303-21;
